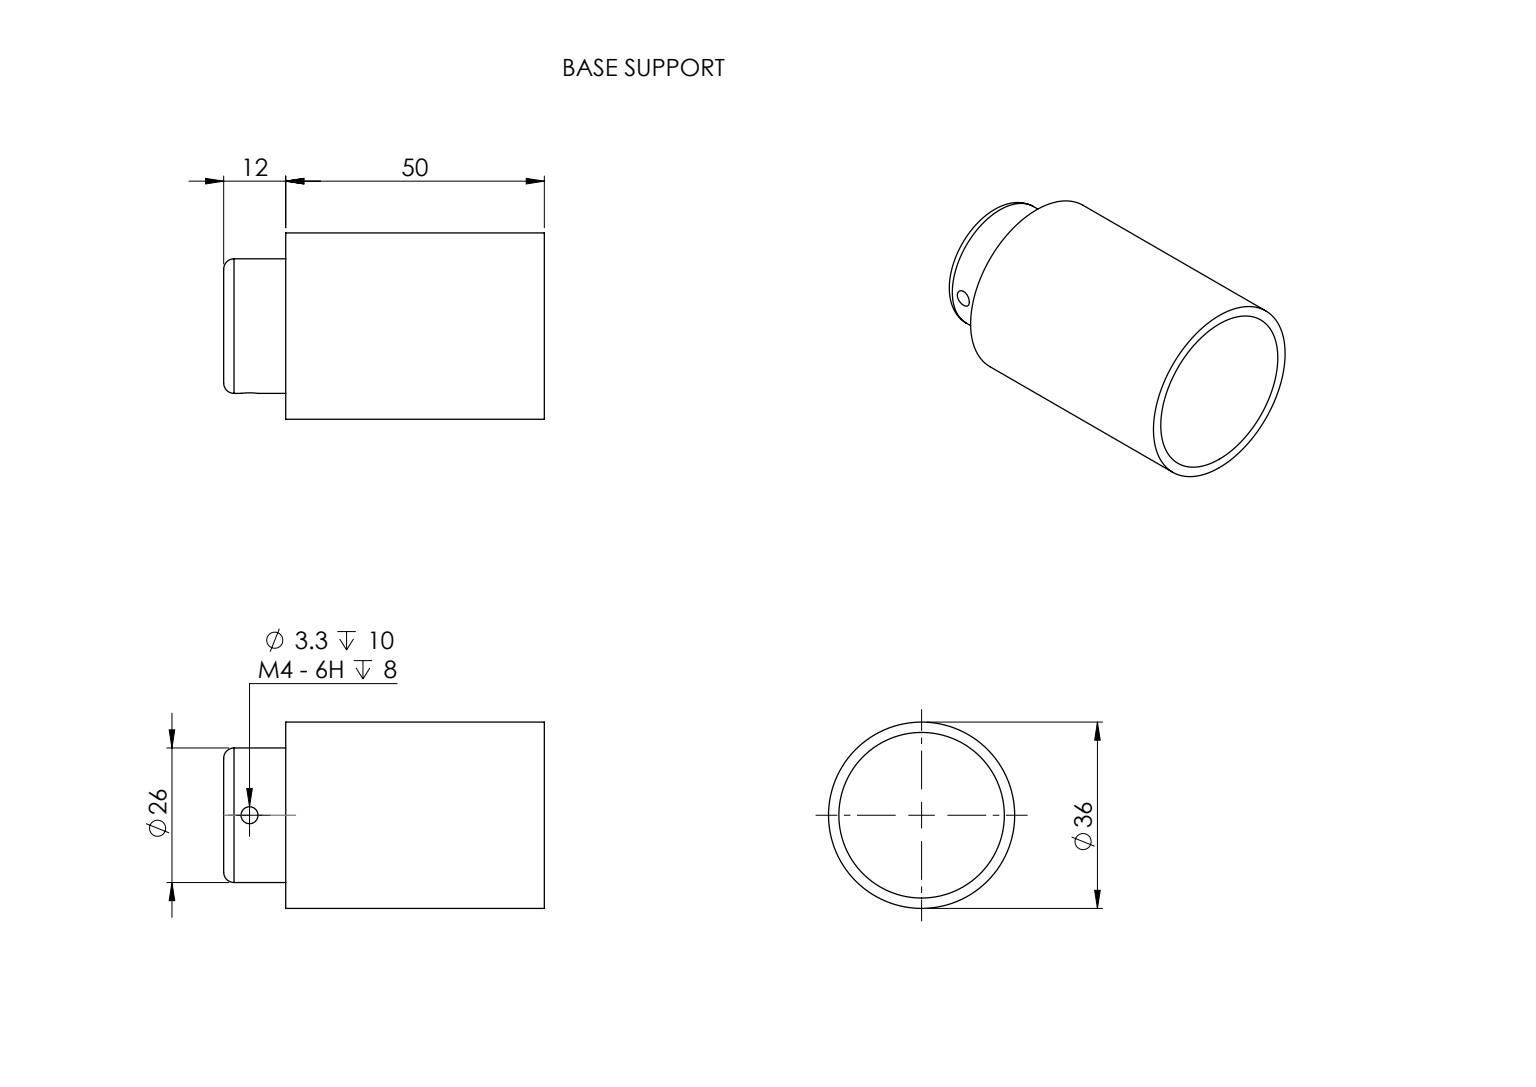
ISO-10303-21;
HEADER;
FILE_DESCRIPTION (('STEP AP214'),
    '1' );
FILE_NAME ('base support.step',
    '2026-10-08T13:22:57',
    ( '' ),
    ( '' ),
    'SwSTEP 2.0',
    'SolidWorks 2026',
    '' );
FILE_SCHEMA (( 'AUTOMOTIVE_DESIGN' ));
ENDSEC;

DATA;
#9=AXIS2_PLACEMENT_3D ( 'NONE', #1726, #4047, #111 ) ;
#21=CARTESIAN_POINT ( 'NONE',  ( -170.0000000000000284, -1.448262861947153525E-15, 0.000000000000000000 ) ) ;
#44=ORIENTED_EDGE ( 'NONE', *, *, #5565, .F. ) ;
#74=EDGE_CURVE ( 'NONE', #951, #9116, #2667, .T. ) ;
#106=CARTESIAN_POINT ( 'NONE',  ( -163.3500000000000796, 0.1091377801384209867, 13.00000000000000178 ) ) ;
#111=DIRECTION ( 'NONE',  ( 1.000000000000000000, 0.000000000000000000, 0.000000000000000000 ) ) ;
#152=FACE_BOUND ( 'NONE', #612, .T. ) ;
#164=AXIS2_PLACEMENT_3D ( 'NONE', #7046, #7979, #7201 ) ;
#171=CIRCLE ( 'NONE', #2486, 11.00000000000000355 ) ;
#181=CIRCLE ( 'NONE', #5941, 18.00000000000000355 ) ;
#189=AXIS2_PLACEMENT_3D ( 'NONE', #6209, #7825, #5544 ) ;
#214=CARTESIAN_POINT ( 'NONE',  ( -163.5173699842553390, 0.7321227054117522837, 12.97975339917165805 ) ) ;
#245=CARTESIAN_POINT ( 'NONE',  ( 0.000000000000000000, 0.000000000000000000, 0.000000000000000000 ) ) ;
#310=EDGE_CURVE ( 'NONE', #9116, #951, #8435, .T. ) ;
#313=EDGE_LOOP ( 'NONE', ( #4589, #4798, #9873, #8476 ) ) ;
#325=CARTESIAN_POINT ( 'NONE',  ( -165.4284909017565326, -1.597016366731424553, 12.90154986763612577 ) ) ;
#348=VECTOR ( 'NONE', #8424, 1000.000000000000000 ) ;
#354=ORIENTED_EDGE ( 'NONE', *, *, #6522, .T. ) ;
#366=LINE ( 'NONE', #6691, #7331 ) ;
#380=DIRECTION ( 'NONE',  ( 0.000000000000000000, 1.000000000000000000, 0.000000000000000000 ) ) ;
#388=ORIENTED_EDGE ( 'NONE', *, *, #1909, .T. ) ;
#394=ADVANCED_FACE ( 'NONE', ( #8448 ), #10092, .T. ) ;
#413=EDGE_LOOP ( 'NONE', ( #2584, #9697, #9041, #6358 ) ) ;
#416=CARTESIAN_POINT ( 'NONE',  ( -166.6500000000000341, -1.532656777835077474E-15, 13.00000000000000355 ) ) ;
#449=AXIS2_PLACEMENT_3D ( 'NONE', #4004, #8752, #7976 ) ;
#451=APPLICATION_CONTEXT ( 'automotive_design' ) ;
#472=DIRECTION ( 'NONE',  ( -1.000000000000000000, -1.387778780781445676E-16, -0.000000000000000000 ) ) ;
#503=VERTEX_POINT ( 'NONE', #9443 ) ;
#520=CARTESIAN_POINT ( 'NONE',  ( -108.0000000000000426, 18.00000000000000355, 0.000000000000000000 ) ) ;
#545=CIRCLE ( 'NONE', #4999, 13.00000000000000533 ) ;
#590=DIRECTION ( 'NONE',  ( -0.000000000000000000, 0.000000000000000000, -1.000000000000000000 ) ) ;
#607=ORIENTED_EDGE ( 'NONE', *, *, #8566, .T. ) ;
#609=ADVANCED_FACE ( 'NONE', ( #8706 ), #801, .F. ) ;
#612=EDGE_LOOP ( 'NONE', ( #1014, #1623 ) ) ;
#656=CARTESIAN_POINT ( 'NONE',  ( -158.0000000000000284, -16.00000000000000355, 0.000000000000000000 ) ) ;
#662=EDGE_LOOP ( 'NONE', ( #7898, #847, #3202, #5619 ) ) ;
#685=LINE ( 'NONE', #2124, #348 ) ;
#726=ORIENTED_EDGE ( 'NONE', *, *, #882, .T. ) ;
#781=FACE_OUTER_BOUND ( 'NONE', #3740, .T. ) ;
#801=CYLINDRICAL_SURFACE ( 'NONE', #164, 15.99999999999999645 ) ;
#830=CARTESIAN_POINT ( 'NONE',  ( -158.0000000000000284, -6.938893903907228378E-15, 0.000000000000000000 ) ) ;
#833=CIRCLE ( 'NONE', #9, 1.649999999999984812 ) ;
#838=CARTESIAN_POINT ( 'NONE',  ( -165.2165827598522867, 1.639280964940008856, 12.89624789671500515 ) ) ;
#847=ORIENTED_EDGE ( 'NONE', *, *, #5286, .T. ) ;
#860=COLOUR_RGB ( '', 0.31764706, 0.68627451, 0.89019608) ;
#882=EDGE_CURVE ( 'NONE', #6987, #9116, #2598, .T. ) ;
#906=CARTESIAN_POINT ( 'NONE',  ( -164.5737606474697543, -1.597621038677511818, 12.90147476577599406 ) ) ;
#943=CARTESIAN_POINT ( 'NONE',  ( -165.4282927514613277, 1.597095956079517709, 12.90154007871212194 ) ) ;
#951=VERTEX_POINT ( 'NONE', #6970 ) ;
#978=ORIENTED_EDGE ( 'NONE', *, *, #8970, .F. ) ;
#992=ADVANCED_FACE ( 'NONE', ( #4599 ), #10132, .F. ) ;
#1004=CIRCLE ( 'NONE', #6592, 11.00000000000000355 ) ;
#1006=CIRCLE ( 'NONE', #2647, 2.000000000000001776 ) ;
#1014=ORIENTED_EDGE ( 'NONE', *, *, #5317, .T. ) ;
#1057=DIRECTION ( 'NONE',  ( -0.000000000000000000, -0.000000000000000000, 1.000000000000000000 ) ) ;
#1095=DIRECTION ( 'NONE',  ( -0.8571673007021101132, 1.049727191138615984E-16, 0.5150380749100580413 ) ) ;
#1118=CARTESIAN_POINT ( 'NONE',  ( -165.0000000000000284, -1.734723475976807094E-15, 3.000000000000002665 ) ) ;
#1188=CARTESIAN_POINT ( 'NONE',  ( -166.6500000000000341, 0.1077421301470921078, 13.00000000000000711 ) ) ;
#1205=CIRCLE ( 'NONE', #4016, 13.00000000000000533 ) ;
#1223=SURFACE_STYLE_FILL_AREA ( #2208 ) ;
#1248=CARTESIAN_POINT ( 'NONE',  ( -168.0000000000000284, -2.363368035607157783E-15, 0.000000000000000000 ) ) ;
#1261=B_SPLINE_CURVE_WITH_KNOTS ( 'NONE', 3,
 ( #8909, #4251, #3421, #4979, #3329, #8862, #1682, #6465, #3471, #2447, #325, #1775, #9539, #5592, #4825, #906, #4928, #4053, #7200, #8075, #6814, #5273, #2846, #2741, #3570, #4300 ),
 .UNSPECIFIED., .F., .F.,
 ( 4, 2, 2, 2, 2, 2, 2, 2, 2, 2, 2, 2, 4 ),
 ( 0.005163858345264566406, 0.005809185821787722637, 0.006454513298310878000, 0.006777177036572426191, 0.007099840774833974383, 0.007422504513095522574, 0.007745168251357070766, 0.008067831989618618957, 0.008390495727880167148, 0.008713159466141713605, 0.009035823204403263531, 0.009681150680926300933, 0.01032647815744933834 ),
 .UNSPECIFIED. ) ;
#1268=( LENGTH_UNIT ( ) NAMED_UNIT ( * ) SI_UNIT ( .MILLI., .METRE. ) );
#1288=CARTESIAN_POINT ( 'NONE',  ( -166.2435802567831331, 1.089887640161022464, 12.95446314200367155 ) ) ;
#1302=CARTESIAN_POINT ( 'NONE',  ( -158.0000000000000284, -6.938893903907228378E-15, 0.000000000000000000 ) ) ;
#1352=( GEOMETRIC_REPRESENTATION_CONTEXT ( 3 ) GLOBAL_UNCERTAINTY_ASSIGNED_CONTEXT ( ( #4119 ) ) GLOBAL_UNIT_ASSIGNED_CONTEXT ( ( #8397, #9910, #4533 ) ) REPRESENTATION_CONTEXT ( 'NONE', 'WORKASPACE' ) );
#1420=DIRECTION ( 'NONE',  ( 0.000000000000000000, -1.000000000000000000, 0.000000000000000000 ) ) ;
#1438=EDGE_LOOP ( 'NONE', ( #8309, #6120, #4912 ) ) ;
#1508=EDGE_CURVE ( 'NONE', #3127, #9396, #1750, .T. ) ;
#1510=ADVANCED_FACE ( 'NONE', ( #9562 ), #7923, .T. ) ;
#1563=AXIS2_PLACEMENT_3D ( 'NONE', #520, #6802, #6597 ) ;
#1613=VERTEX_POINT ( 'NONE', #2001 ) ;
#1616=CARTESIAN_POINT ( 'NONE',  ( -168.0000000000000284, -2.363368035607157783E-15, 0.000000000000000000 ) ) ;
#1623=ORIENTED_EDGE ( 'NONE', *, *, #5748, .T. ) ;
#1637=CARTESIAN_POINT ( 'NONE',  ( -170.0000000000000284, -1.448262861947153525E-15, 0.000000000000000000 ) ) ;
#1666=FACE_OUTER_BOUND ( 'NONE', #313, .T. ) ;
#1676=AXIS2_PLACEMENT_3D ( 'NONE', #7871, #8656, #7781 ) ;
#1682=CARTESIAN_POINT ( 'NONE',  ( -166.0067307485407184, -1.311714535335565923, 12.93379411699749681 ) ) ;
#1720=CARTESIAN_POINT ( 'NONE',  ( -163.4027093359710534, 0.4274795813385452448, 12.99339846045314850 ) ) ;
#1726=CARTESIAN_POINT ( 'NONE',  ( -165.0000000000000284, -1.734723475976807094E-15, 3.000000000000002665 ) ) ;
#1750=LINE ( 'NONE', #5814, #7591 ) ;
#1763=LINE ( 'NONE', #9577, #3701 ) ;
#1775=CARTESIAN_POINT ( 'NONE',  ( -165.2175649311437837, -1.639125141419205622, 12.89626763964974465 ) ) ;
#1783=EDGE_CURVE ( 'NONE', #503, #6536, #171, .T. ) ;
#1826=AXIS2_PLACEMENT_3D ( 'NONE', #4668, #5385, #3735 ) ;
#1863=ORIENTED_EDGE ( 'NONE', *, *, #1508, .T. ) ;
#1866=CARTESIAN_POINT ( 'NONE',  ( -164.7839123519666487, 1.649920478573665195, 12.89487349378784664 ) ) ;
#1870=EDGE_CURVE ( 'NONE', #5718, #951, #10115, .T. ) ;
#1871=DIRECTION ( 'NONE',  ( 0.000000000000000000, -1.000000000000000000, 0.000000000000000000 ) ) ;
#1881=DIRECTION ( 'NONE',  ( -5.603403109029596495E-32, -1.224646799147353207E-16, 1.000000000000000000 ) ) ;
#1905=ORIENTED_EDGE ( 'NONE', *, *, #6467, .T. ) ;
#1909=EDGE_CURVE ( 'NONE', #6987, #5718, #9429, .T. ) ;
#1982=ORIENTED_EDGE ( 'NONE', *, *, #310, .T. ) ;
#1988=DIRECTION ( 'NONE',  ( -4.575525868300071581E-16, -1.000000000000000000, 0.000000000000000000 ) ) ;
#1995=VECTOR ( 'NONE', #4731, 1000.000000000000000 ) ;
#2001=CARTESIAN_POINT ( 'NONE',  ( -158.0000000000000284, -13.00000000000001066, 1.592040838891559884E-15 ) ) ;
#2014=CARTESIAN_POINT ( 'NONE',  ( -166.5969417738770346, 0.4288646725500943613, 12.99335536005336955 ) ) ;
#2060=EDGE_CURVE ( 'NONE', #6536, #503, #1004, .T. ) ;
#2065=CARTESIAN_POINT ( 'NONE',  ( -170.0000000000000284, 11.00000000000000178, 1.469576158976824539E-15 ) ) ;
#2097=( NAMED_UNIT ( * ) SI_UNIT ( $, .STERADIAN. ) SOLID_ANGLE_UNIT ( ) );
#2118=LINE ( 'NONE', #9875, #8996 ) ;
#2124=CARTESIAN_POINT ( 'NONE',  ( -158.0000000000000284, -13.00000000000001066, 1.592040838891559490E-15 ) ) ;
#2144=CARTESIAN_POINT ( 'NONE',  ( -158.0000000000000284, -6.938893903907228378E-15, 0.000000000000000000 ) ) ;
#2145=FACE_OUTER_BOUND ( 'NONE', #4650, .T. ) ;
#2151=SURFACE_STYLE_USAGE ( .BOTH. , #8508 ) ;
#2185=DIRECTION ( 'NONE',  ( -0.000000000000000000, -0.000000000000000000, 1.000000000000000000 ) ) ;
#2202=DIRECTION ( 'NONE',  ( 0.000000000000000000, -1.000000000000000000, 0.000000000000000000 ) ) ;
#2208=FILL_AREA_STYLE ('',( #6781 ) ) ;
#2239=FACE_OUTER_BOUND ( 'NONE', #413, .T. ) ;
#2264=ADVANCED_FACE ( 'NONE', ( #8085 ), #5129, .F. ) ;
#2310=DIRECTION ( 'NONE',  ( 0.000000000000000000, -1.000000000000000000, 0.000000000000000000 ) ) ;
#2359=CIRCLE ( 'NONE', #2542, 13.00000000000000355 ) ;
#2364=SHAPE_DEFINITION_REPRESENTATION ( #5902, #5586 ) ;
#2435=CARTESIAN_POINT ( 'NONE',  ( -165.8275777035124747, 1.431488817417934101, 12.92108529057806798 ) ) ;
#2447=CARTESIAN_POINT ( 'NONE',  ( -165.5332536431789094, -1.565195349311612416, 12.90549919778201904 ) ) ;
#2477=VECTOR ( 'NONE', #8016, 1000.000000000000000 ) ;
#2482=CARTESIAN_POINT ( 'NONE',  ( -163.5680690899785930, 0.8268589710946947502, 12.97398861359800115 ) ) ;
#2486=AXIS2_PLACEMENT_3D ( 'NONE', #1637, #10163, #4736 ) ;
#2498=CARTESIAN_POINT ( 'NONE',  ( -158.0000000000000284, -6.938893903907228378E-15, 0.000000000000000000 ) ) ;
#2524=VERTEX_POINT ( 'NONE', #9898 ) ;
#2542=AXIS2_PLACEMENT_3D ( 'NONE', #1616, #4613, #6093 ) ;
#2584=ORIENTED_EDGE ( 'NONE', *, *, #9584, .F. ) ;
#2595=FACE_BOUND ( 'NONE', #7310, .T. ) ;
#2598=LINE ( 'NONE', #3472, #5924 ) ;
#2630=FACE_OUTER_BOUND ( 'NONE', #9178, .T. ) ;
#2643=DIRECTION ( 'NONE',  ( 1.000000000000000000, -4.575525868300071581E-16, -0.000000000000000000 ) ) ;
#2647=AXIS2_PLACEMENT_3D ( 'NONE', #3893, #590, #4517 ) ;
#2667=CIRCLE ( 'NONE', #8620, 18.00000000000000355 ) ;
#2681=CYLINDRICAL_SURFACE ( 'NONE', #7208, 18.00000000000000355 ) ;
#2695=CARTESIAN_POINT ( 'NONE',  ( -168.0000000000000284, 13.00000000000000178, 0.000000000000000000 ) ) ;
#2705=ORIENTED_EDGE ( 'NONE', *, *, #2060, .F. ) ;
#2734=FACE_OUTER_BOUND ( 'NONE', #1438, .T. ) ;
#2741=CARTESIAN_POINT ( 'NONE',  ( -163.3939431418218646, -0.4350255360096275670, 12.99423751676100558 ) ) ;
#2781=EDGE_CURVE ( 'NONE', #9967, #8413, #8938, .T. ) ;
#2846=CARTESIAN_POINT ( 'NONE',  ( -163.5589117782047595, -0.8318236505920658663, 12.97488054948080993 ) ) ;
#2886=FACE_OUTER_BOUND ( 'NONE', #8049, .T. ) ;
#2903=EDGE_CURVE ( 'NONE', #10190, #9396, #6449, .T. ) ;
#2943=DIRECTION ( 'NONE',  ( 1.000000000000000000, 0.000000000000000000, 0.000000000000000000 ) ) ;
#2949=CARTESIAN_POINT ( 'NONE',  ( -166.6500000000000341, -1.532656777835077474E-15, 13.00000000000000355 ) ) ;
#2953=CARTESIAN_POINT ( 'NONE',  ( -108.0000000000000426, 15.99999999999999289, 1.959434878635764737E-15 ) ) ;
#3094=CYLINDRICAL_SURFACE ( 'NONE', #3255, 1.649999999999984812 ) ;
#3122=CARTESIAN_POINT ( 'NONE',  ( -168.0000000000000284, -13.00000000000000533, 1.592040838891559490E-15 ) ) ;
#3127=VERTEX_POINT ( 'NONE', #6508 ) ;
#3143=ADVANCED_FACE ( 'NONE', ( #2595, #5791 ), #3419, .T. ) ;
#3152=STYLED_ITEM ( 'NONE', ( #9506 ), #7057 ) ;
#3153=AXIS2_PLACEMENT_3D ( 'NONE', #5901, #9077, #1988 ) ;
#3161=( GEOMETRIC_REPRESENTATION_CONTEXT ( 3 ) GLOBAL_UNCERTAINTY_ASSIGNED_CONTEXT ( ( #8141 ) ) GLOBAL_UNIT_ASSIGNED_CONTEXT ( ( #1268, #9235, #2097 ) ) REPRESENTATION_CONTEXT ( 'NONE', 'WORKASPACE' ) );
#3190=AXIS2_PLACEMENT_3D ( 'NONE', #5290, #5144, #8391 ) ;
#3202=ORIENTED_EDGE ( 'NONE', *, *, #1783, .F. ) ;
#3204=EDGE_CURVE ( 'NONE', #9396, #6730, #9685, .T. ) ;
#3218=LINE ( 'NONE', #4096, #2477 ) ;
#3255=AXIS2_PLACEMENT_3D ( 'NONE', #8526, #3774, #6906 ) ;
#3272=DIRECTION ( 'NONE',  ( -1.000000000000000000, -1.387778780781445676E-16, -0.000000000000000000 ) ) ;
#3310=AXIS2_PLACEMENT_3D ( 'NONE', #10146, #8494, #1420 ) ;
#3329=CARTESIAN_POINT ( 'NONE',  ( -166.3194911921033849, -1.013757292147143385, 12.96131341066429954 ) ) ;
#3342=FILL_AREA_STYLE_COLOUR ( '', #7114 ) ;
#3394=CARTESIAN_POINT ( 'NONE',  ( -166.6500000000000341, -1.532656754117495520E-15, 3.000000000000002665 ) ) ;
#3397=CARTESIAN_POINT ( 'NONE',  ( -168.0000000000000284, -2.363368035607170010E-15, 0.000000000000000000 ) ) ;
#3411=CARTESIAN_POINT ( 'NONE',  ( -164.1695521934695989, 1.441888585351695395, 12.92005519273647707 ) ) ;
#3419=CYLINDRICAL_SURFACE ( 'NONE', #449, 13.00000000000000355 ) ;
#3421=CARTESIAN_POINT ( 'NONE',  ( -166.6066941517921123, -0.4327006227615173839, 12.99431788236279139 ) ) ;
#3445=EDGE_LOOP ( 'NONE', ( #8575, #3826, #7606, #9478 ) ) ;
#3451=ORIENTED_EDGE ( 'NONE', *, *, #5975, .F. ) ;
#3468=VERTEX_POINT ( 'NONE', #2695 ) ;
#3471=CARTESIAN_POINT ( 'NONE',  ( -165.7329923747223859, -1.482200427765804296, 12.91529434110542240 ) ) ;
#3472=CARTESIAN_POINT ( 'NONE',  ( -158.0000000000000284, -18.00000000000001066, 0.000000000000000000 ) ) ;
#3565=CARTESIAN_POINT ( 'NONE',  ( -108.0000000000000426, 0.000000000000000000, 0.000000000000000000 ) ) ;
#3570=CARTESIAN_POINT ( 'NONE',  ( -163.3500000000000796, -0.2182232076591351377, 13.00000000000000533 ) ) ;
#3598=ORIENTED_EDGE ( 'NONE', *, *, #1870, .F. ) ;
#3646=ADVANCED_FACE ( 'NONE', ( #2630 ), #2681, .T. ) ;
#3689=ORIENTED_EDGE ( 'NONE', *, *, #3204, .F. ) ;
#3701=VECTOR ( 'NONE', #4141, 1000.000000000000000 ) ;
#3709=CARTESIAN_POINT ( 'NONE',  ( -108.0000000000000426, -18.00000000000000355, 0.000000000000000000 ) ) ;
#3735=DIRECTION ( 'NONE',  ( 0.000000000000000000, -1.000000000000000000, 0.000000000000000000 ) ) ;
#3740=EDGE_LOOP ( 'NONE', ( #1982, #8387 ) ) ;
#3774=DIRECTION ( 'NONE',  ( -0.000000000000000000, -0.000000000000000000, 1.000000000000000000 ) ) ;
#3826=ORIENTED_EDGE ( 'NONE', *, *, #9652, .T. ) ;
#3836=ADVANCED_FACE ( 'NONE', ( #5258 ), #3094, .F. ) ;
#3842=CARTESIAN_POINT ( 'NONE',  ( -156.0000000000000284, -16.00000000000000711, 0.000000000000000000 ) ) ;
#3893=CARTESIAN_POINT ( 'NONE',  ( -168.0000000000000284, -11.00000000000000533, 0.000000000000000000 ) ) ;
#3977=AXIS2_PLACEMENT_3D ( 'NONE', #1118, #5704, #7363 ) ;
#3986=PLANE ( 'NONE',  #7782 ) ;
#3988=AXIS2_PLACEMENT_3D ( 'NONE', #5116, #2185, #2943 ) ;
#3995=AXIS2_PLACEMENT_3D ( 'NONE', #245, #8930, #7419 ) ;
#4004=CARTESIAN_POINT ( 'NONE',  ( -158.0000000000000284, -6.938893903907228378E-15, 0.000000000000000000 ) ) ;
#4016=AXIS2_PLACEMENT_3D ( 'NONE', #1302, #9216, #380 ) ;
#4044=CARTESIAN_POINT ( 'NONE',  ( -158.0000000000000284, -6.938893903907228378E-15, 0.000000000000000000 ) ) ;
#4047=DIRECTION ( 'NONE',  ( -0.000000000000000000, -0.000000000000000000, 1.000000000000000000 ) ) ;
#4053=CARTESIAN_POINT ( 'NONE',  ( -164.2691053559693728, -1.483232571104735609, 12.91517534017533109 ) ) ;
#4089=CARTESIAN_POINT ( 'NONE',  ( -165.5312037683856943, 1.565894570282060583, 12.90541399993123228 ) ) ;
#4096=CARTESIAN_POINT ( 'NONE',  ( -158.0000000000000284, 15.99999999999998934, 1.959434878635764737E-15 ) ) ;
#4119=UNCERTAINTY_MEASURE_WITH_UNIT (LENGTH_MEASURE( 1.000000000000000082E-05 ), #8397, 'distance_accuracy_value', 'NONE');
#4141=DIRECTION ( 'NONE',  ( -0.000000000000000000, -0.000000000000000000, 1.000000000000000000 ) ) ;
#4144=AXIS2_PLACEMENT_3D ( 'NONE', #5292, #8449, #2202 ) ;
#4153=DIRECTION ( 'NONE',  ( 0.000000000000000000, -1.000000000000000000, -1.224646799147353454E-16 ) ) ;
#4192=DIRECTION ( 'NONE',  ( 1.000000000000000000, -4.575525868300071581E-16, -0.000000000000000000 ) ) ;
#4235=DIRECTION ( 'NONE',  ( 1.000000000000000000, -4.575525868300071581E-16, -0.000000000000000000 ) ) ;
#4251=CARTESIAN_POINT ( 'NONE',  ( -166.6500000000000057, -0.2154325771598549211, 13.00000000000000533 ) ) ;
#4275=EDGE_LOOP ( 'NONE', ( #5969, #1863, #9950 ) ) ;
#4300=CARTESIAN_POINT ( 'NONE',  ( -163.3500000000000512, -1.154202410357457390E-14, 13.00000000000000355 ) ) ;
#4301=VECTOR ( 'NONE', #6221, 1000.000000000000000 ) ;
#4312=ORIENTED_EDGE ( 'NONE', *, *, #74, .F. ) ;
#4337=CARTESIAN_POINT ( 'NONE',  ( -166.4312272284851986, 0.8280293812990602298, 12.97391163473193387 ) ) ;
#4379=ORIENTED_EDGE ( 'NONE', *, *, #1870, .T. ) ;
#4454=DIRECTION ( 'NONE',  ( 1.000000000000000000, -4.575525868300071581E-16, -0.000000000000000000 ) ) ;
#4486=STYLED_ITEM ( 'NONE', ( #5201 ), #8958 ) ;
#4517=DIRECTION ( 'NONE',  ( -1.000000000000000000, 0.000000000000000000, 0.000000000000000000 ) ) ;
#4533=( NAMED_UNIT ( * ) SI_UNIT ( $, .STERADIAN. ) SOLID_ANGLE_UNIT ( ) );
#4539=ORIENTED_EDGE ( 'NONE', *, *, #9349, .F. ) ;
#4541=DIRECTION ( 'NONE',  ( 0.000000000000000000, -1.000000000000000000, 0.000000000000000000 ) ) ;
#4573=EDGE_LOOP ( 'NONE', ( #7823, #3451, #5167, #2705 ) ) ;
#4585=SHAPE_REPRESENTATION_RELATIONSHIP ( 'NONE' , 'NONE' ,  #5586, #8958 ) ;
#4589=ORIENTED_EDGE ( 'NONE', *, *, #9652, .F. ) ;
#4599=FACE_OUTER_BOUND ( 'NONE', #9240, .T. ) ;
#4607=CARTESIAN_POINT ( 'NONE',  ( -156.0000000000000284, -6.938893903907228378E-15, 0.000000000000000000 ) ) ;
#4613=DIRECTION ( 'NONE',  ( 1.000000000000000000, -4.575525868300071581E-16, -0.000000000000000000 ) ) ;
#4650=EDGE_LOOP ( 'NONE', ( #388, #4379, #5159, #4762 ) ) ;
#4661=ORIENTED_EDGE ( 'NONE', *, *, #1909, .F. ) ;
#4668=CARTESIAN_POINT ( 'NONE',  ( -158.0000000000000284, -6.938893903907228378E-15, 0.000000000000000000 ) ) ;
#4731=DIRECTION ( 'NONE',  ( -1.000000000000000000, -1.387778780781445676E-16, -0.000000000000000000 ) ) ;
#4736=DIRECTION ( 'NONE',  ( 0.000000000000000000, -1.000000000000000000, 0.000000000000000000 ) ) ;
#4739=SURFACE_SIDE_STYLE ('',( #4940 ) ) ;
#4762=ORIENTED_EDGE ( 'NONE', *, *, #882, .F. ) ;
#4782=AXIS2_PLACEMENT_3D ( 'NONE', #2144, #5349, #5291 ) ;
#4789=AXIS2_PLACEMENT_3D ( 'NONE', #3397, #5617, #8837 ) ;
#4798=ORIENTED_EDGE ( 'NONE', *, *, #5975, .T. ) ;
#4814=ADVANCED_FACE ( 'NONE', ( #9900 ), #10001, .F. ) ;
#4815=CARTESIAN_POINT ( 'NONE',  ( -163.9856078553142709, 1.318997900831586856, 12.93381406529030642 ) ) ;
#4825=CARTESIAN_POINT ( 'NONE',  ( -164.7848126586117985, -1.639441178260655052, 12.89622722885275152 ) ) ;
#4842=AXIS2_PLACEMENT_3D ( 'NONE', #21, #6993, #8501 ) ;
#4866=CARTESIAN_POINT ( 'NONE',  ( -163.7574652328086131, 1.090948703523729746, 12.95436823472124566 ) ) ;
#4912=ORIENTED_EDGE ( 'NONE', *, *, #2903, .T. ) ;
#4928=CARTESIAN_POINT ( 'NONE',  ( -164.4688726891355088, -1.565914946704515254, 12.90541139627661593 ) ) ;
#4940=SURFACE_STYLE_FILL_AREA ( #9657 ) ;
#4964=CIRCLE ( 'NONE', #3310, 16.00000000000000000 ) ;
#4979=CARTESIAN_POINT ( 'NONE',  ( -166.4422304502845407, -0.8298597800914565559, 12.97500904825187540 ) ) ;
#4981=ADVANCED_FACE ( 'NONE', ( #5348 ), #5499, .T. ) ;
#4986=CLOSED_SHELL ( 'NONE', ( #3836, #9463, #394, #3143, #7435, #8404, #992, #609, #6555, #3646, #9871, #6343, #4981, #1510, #2264, #4814 ) ) ;
#4999=AXIS2_PLACEMENT_3D ( 'NONE', #2498, #2643, #8126 ) ;
#5014=CARTESIAN_POINT ( 'NONE',  ( -165.1071317273496959, 1.650039592648423259, 12.89485825219862569 ) ) ;
#5066=CARTESIAN_POINT ( 'NONE',  ( -163.3500000000000512, -1.734723475976807094E-15, 3.000000000000002665 ) ) ;
#5087=PRODUCT ( 'base support', 'base support', '', ( #10170 ) ) ;
#5088=B_SPLINE_CURVE_WITH_KNOTS ( 'NONE', 3,
 ( #7291, #106, #8802, #1720, #6351, #214, #2482, #5636, #4866, #4815, #3411, #6547, #1866, #5014, #838, #943, #4089, #9529, #2435, #5581, #7965, #1288, #7387, #4337, #7440, #9104, #2014, #8265, #1188, #416 ),
 .UNSPECIFIED., .F., .F.,
 ( 4, 2, 2, 2, 2, 2, 2, 2, 2, 2, 2, 2, 2, 2, 4 ),
 ( 6.815973429434667561E-18, 0.0003227411465790211431, 0.0006454822931580354558, 0.0009682234397370497684, 0.001290964586316063973, 0.001936446879474092598, 0.002581929172632121440, 0.002904670319211177278, 0.003227411465790232682, 0.003550152612369288519, 0.003872893758948343923, 0.004195634905527399761, 0.004518376052106455598, 0.004841117198685510568, 0.005163858345264566406 ),
 .UNSPECIFIED. ) ;
#5116=CARTESIAN_POINT ( 'NONE',  ( -165.0000000000000284, -1.734723475976807094E-15, 3.000000000000002665 ) ) ;
#5129=CONICAL_SURFACE ( 'NONE', #3977, 1.649999999999984812, 1.029744258676650093 ) ;
#5144=DIRECTION ( 'NONE',  ( -0.000000000000000000, -0.000000000000000000, 1.000000000000000000 ) ) ;
#5159=ORIENTED_EDGE ( 'NONE', *, *, #310, .F. ) ;
#5167=ORIENTED_EDGE ( 'NONE', *, *, #8383, .T. ) ;
#5201=PRESENTATION_STYLE_ASSIGNMENT (( #2151 ) ) ;
#5216=PLANE ( 'NONE',  #1563 ) ;
#5249=CARTESIAN_POINT ( 'NONE',  ( -158.0000000000000284, -6.938893903907228378E-15, 0.000000000000000000 ) ) ;
#5258=FACE_OUTER_BOUND ( 'NONE', #9916, .T. ) ;
#5273=CARTESIAN_POINT ( 'NONE',  ( -163.6819620139764595, -1.015622990690433936, 12.96116402481652408 ) ) ;
#5286=EDGE_CURVE ( 'NONE', #3468, #6536, #5331, .T. ) ;
#5288=CIRCLE ( 'NONE', #9770, 16.00000000000000000 ) ;
#5290=CARTESIAN_POINT ( 'NONE',  ( -165.0000000000000284, -1.734723475976807094E-15, 13.00000000000000355 ) ) ;
#5291=DIRECTION ( 'NONE',  ( 0.000000000000000000, -1.000000000000000000, 0.000000000000000000 ) ) ;
#5292=CARTESIAN_POINT ( 'NONE',  ( -158.0000000000000284, -6.938893903907228378E-15, 0.000000000000000000 ) ) ;
#5317=EDGE_CURVE ( 'NONE', #2524, #1613, #545, .T. ) ;
#5331=CIRCLE ( 'NONE', #6974, 2.000000000000000000 ) ;
#5348=FACE_OUTER_BOUND ( 'NONE', #8939, .T. ) ;
#5349=DIRECTION ( 'NONE',  ( -1.000000000000000000, -1.387778780781445676E-16, -0.000000000000000000 ) ) ;
#5385=DIRECTION ( 'NONE',  ( -1.000000000000000000, -1.387778780781445676E-16, -0.000000000000000000 ) ) ;
#5418=ORIENTED_EDGE ( 'NONE', *, *, #2060, .T. ) ;
#5499=PLANE ( 'NONE',  #4842 ) ;
#5509=DIRECTION ( 'NONE',  ( -1.000000000000000000, 4.575525868300071581E-16, 0.000000000000000000 ) ) ;
#5531=EDGE_LOOP ( 'NONE', ( #8199, #8633 ) ) ;
#5544=DIRECTION ( 'NONE',  ( 1.000000000000000000, 0.000000000000000000, 0.000000000000000000 ) ) ;
#5556=CARTESIAN_POINT ( 'NONE',  ( -158.0000000000000284, 17.99999999999999645, 2.204364238465235822E-15 ) ) ;
#5565=EDGE_CURVE ( 'NONE', #5950, #6730, #1261, .T. ) ;
#5581=CARTESIAN_POINT ( 'NONE',  ( -166.0062384261120769, 1.312070622931204689, 12.93375722677777340 ) ) ;
#5586=SHAPE_REPRESENTATION ( 'base support', ( #3995 ), #3161 ) ;
#5592=CARTESIAN_POINT ( 'NONE',  ( -164.8920828308066859, -1.650077165904365373, 12.89485344440482173 ) ) ;
#5604=PRODUCT_DEFINITION ( 'UNKNOWN', '', #7888, #7116 ) ;
#5617=DIRECTION ( 'NONE',  ( -1.000000000000000000, 4.575525868300071581E-16, 0.000000000000000000 ) ) ;
#5619=ORIENTED_EDGE ( 'NONE', *, *, #8383, .F. ) ;
#5629=DIRECTION ( 'NONE',  ( 1.000000000000000000, 1.387778780781445676E-16, 0.000000000000000000 ) ) ;
#5636=CARTESIAN_POINT ( 'NONE',  ( -163.6878309682295765, 1.006148260057784238, 12.96131713918894235 ) ) ;
#5704=DIRECTION ( 'NONE',  ( -0.000000000000000000, -0.000000000000000000, 1.000000000000000000 ) ) ;
#5714=DIRECTION ( 'NONE',  ( 0.8571673007021101132, 0.000000000000000000, 0.5150380749100580413 ) ) ;
#5718=VERTEX_POINT ( 'NONE', #7669 ) ;
#5748=EDGE_CURVE ( 'NONE', #1613, #2524, #1205, .T. ) ;
#5756=UNCERTAINTY_MEASURE_WITH_UNIT (LENGTH_MEASURE( 1.000000000000000082E-05 ), #7886, 'distance_accuracy_value', 'NONE');
#5778=DIRECTION ( 'NONE',  ( 0.000000000000000000, -1.000000000000000000, 0.000000000000000000 ) ) ;
#5791=FACE_OUTER_BOUND ( 'NONE', #3445, .T. ) ;
#5814=CARTESIAN_POINT ( 'NONE',  ( -163.3500000000000512, -1.734723475976807094E-15, 3.000000000000002665 ) ) ;
#5870=VECTOR ( 'NONE', #1057, 1000.000000000000000 ) ;
#5874=CARTESIAN_POINT ( 'NONE',  ( -158.0000000000000284, -6.938893903907228378E-15, 0.000000000000000000 ) ) ;
#5895=ORIENTED_EDGE ( 'NONE', *, *, #6467, .F. ) ;
#5901=CARTESIAN_POINT ( 'NONE',  ( -168.0000000000000284, -2.363368035607170010E-15, 0.000000000000000000 ) ) ;
#5902=PRODUCT_DEFINITION_SHAPE ( 'NONE', 'NONE',  #5604 ) ;
#5911=EDGE_CURVE ( 'NONE', #3468, #7869, #7670, .T. ) ;
#5924=VECTOR ( 'NONE', #3272, 1000.000000000000000 ) ;
#5941=AXIS2_PLACEMENT_3D ( 'NONE', #3565, #7496, #1871 ) ;
#5950=VERTEX_POINT ( 'NONE', #2949 ) ;
#5969=ORIENTED_EDGE ( 'NONE', *, *, #6565, .F. ) ;
#5975=EDGE_CURVE ( 'NONE', #7869, #3468, #2359, .T. ) ;
#5977=VERTEX_POINT ( 'NONE', #3842 ) ;
#5999=EDGE_LOOP ( 'NONE', ( #7068, #8364, #9837, #607 ) ) ;
#6032=CARTESIAN_POINT ( 'NONE',  ( -108.0000000000000426, 0.000000000000000000, 0.000000000000000000 ) ) ;
#6054=CYLINDRICAL_SURFACE ( 'NONE', #4144, 18.00000000000000355 ) ;
#6093=DIRECTION ( 'NONE',  ( 0.000000000000000000, -1.000000000000000000, 0.000000000000000000 ) ) ;
#6120=ORIENTED_EDGE ( 'NONE', *, *, #6565, .T. ) ;
#6209=CARTESIAN_POINT ( 'NONE',  ( -165.0000000000000284, -1.734723475976807094E-15, 3.000000000000002665 ) ) ;
#6221=DIRECTION ( 'NONE',  ( -1.000000000000000000, -1.387778780781445676E-16, -0.000000000000000000 ) ) ;
#6324=SURFACE_STYLE_USAGE ( .BOTH. , #4739 ) ;
#6335=ORIENTED_EDGE ( 'NONE', *, *, #5565, .T. ) ;
#6343=ADVANCED_FACE ( 'NONE', ( #1666 ), #7140, .T. ) ;
#6344=DIRECTION ( 'NONE',  ( -1.387778780781445676E-16, 1.000000000000000000, 0.000000000000000000 ) ) ;
#6351=CARTESIAN_POINT ( 'NONE',  ( -163.4344937688939865, 0.5323397972486557661, 12.98948098652724603 ) ) ;
#6358=ORIENTED_EDGE ( 'NONE', *, *, #7789, .F. ) ;
#6410=CARTESIAN_POINT ( 'NONE',  ( -163.3500000000000512, -1.734723475976807094E-15, 13.00000000000000355 ) ) ;
#6449=CIRCLE ( 'NONE', #189, 1.649999999999984812 ) ;
#6465=CARTESIAN_POINT ( 'NONE',  ( -165.8276565213533900, -1.431463064465520851, 12.92108891611541566 ) ) ;
#6467=EDGE_CURVE ( 'NONE', #10190, #5950, #1763, .T. ) ;
#6508=CARTESIAN_POINT ( 'NONE',  ( -165.0000000000000284, -1.734723475976807094E-15, 2.008579978604527305 ) ) ;
#6522=EDGE_CURVE ( 'NONE', #6730, #5950, #5088, .T. ) ;
#6536=VERTEX_POINT ( 'NONE', #2065 ) ;
#6547=CARTESIAN_POINT ( 'NONE',  ( -164.5666002992762458, 1.606502708168054738, 12.90062083485027777 ) ) ;
#6555=ADVANCED_FACE ( 'NONE', ( #2886, #8160 ), #5216, .F. ) ;
#6565=EDGE_CURVE ( 'NONE', #3127, #10190, #366, .T. ) ;
#6592=AXIS2_PLACEMENT_3D ( 'NONE', #8617, #5509, #7795 ) ;
#6597=DIRECTION ( 'NONE',  ( 1.387778780781445676E-16, -1.000000000000000000, 0.000000000000000000 ) ) ;
#6620=EDGE_CURVE ( 'NONE', #3468, #2524, #2118, .T. ) ;
#6633=ORIENTED_EDGE ( 'NONE', *, *, #9306, .F. ) ;
#6642=EDGE_LOOP ( 'NONE', ( #5895, #978, #9726, #354 ) ) ;
#6649=CARTESIAN_POINT ( 'NONE',  ( -156.0000000000000284, -6.661338147750945553E-15, 0.000000000000000000 ) ) ;
#6691=CARTESIAN_POINT ( 'NONE',  ( -166.6500000000000341, -1.532656754117495520E-15, 3.000000000000002665 ) ) ;
#6730=VERTEX_POINT ( 'NONE', #9158 ) ;
#6744=DIRECTION ( 'NONE',  ( 0.000000000000000000, -1.000000000000000000, 0.000000000000000000 ) ) ;
#6756=AXIS2_PLACEMENT_3D ( 'NONE', #6032, #9212, #9367 ) ;
#6781=FILL_AREA_STYLE_COLOUR ( '', #860 ) ;
#6787=ORIENTED_EDGE ( 'NONE', *, *, #2903, .F. ) ;
#6802=DIRECTION ( 'NONE',  ( -1.000000000000000000, -1.387778780781445676E-16, 0.000000000000000000 ) ) ;
#6814=CARTESIAN_POINT ( 'NONE',  ( -163.9101340986164246, -1.243481348857424562, 12.94061705906631055 ) ) ;
#6851=VERTEX_POINT ( 'NONE', #9258 ) ;
#6906=DIRECTION ( 'NONE',  ( 1.000000000000000000, 0.000000000000000000, 0.000000000000000000 ) ) ;
#6970=CARTESIAN_POINT ( 'NONE',  ( -158.0000000000000284, 17.99999999999999645, 2.204364238465235822E-15 ) ) ;
#6974=AXIS2_PLACEMENT_3D ( 'NONE', #8968, #1881, #4153 ) ;
#6987=VERTEX_POINT ( 'NONE', #3709 ) ;
#6993=DIRECTION ( 'NONE',  ( -1.000000000000000000, 4.575525868300071581E-16, 0.000000000000000000 ) ) ;
#7046=CARTESIAN_POINT ( 'NONE',  ( -158.0000000000000284, -6.938893903907228378E-15, 0.000000000000000000 ) ) ;
#7057=MANIFOLD_SOLID_BREP ( 'M4 Tapped Hole1', #4986 ) ;
#7068=ORIENTED_EDGE ( 'NONE', *, *, #8641, .F. ) ;
#7098=LINE ( 'NONE', #656, #1995 ) ;
#7114=COLOUR_RGB ( '', 0.31764706, 0.68627451, 0.89019608) ;
#7116=PRODUCT_DEFINITION_CONTEXT ( 'detailed design', #451, 'design' ) ;
#7140=CYLINDRICAL_SURFACE ( 'NONE', #9321, 13.00000000000000355 ) ;
#7200=CARTESIAN_POINT ( 'NONE',  ( -164.1743453116437763, -1.432625545945890311, 12.92095975507885441 ) ) ;
#7201=DIRECTION ( 'NONE',  ( 0.000000000000000000, -1.000000000000000000, 0.000000000000000000 ) ) ;
#7208=AXIS2_PLACEMENT_3D ( 'NONE', #5874, #9930, #5778 ) ;
#7275=ORIENTED_EDGE ( 'NONE', *, *, #6522, .F. ) ;
#7291=CARTESIAN_POINT ( 'NONE',  ( -163.3500000000000512, -1.154202410357457390E-14, 13.00000000000000355 ) ) ;
#7310=EDGE_LOOP ( 'NONE', ( #7275, #44 ) ) ;
#7331=VECTOR ( 'NONE', #1095, 999.9999999999998863 ) ;
#7363=DIRECTION ( 'NONE',  ( 1.000000000000000000, 0.000000000000000000, 0.000000000000000000 ) ) ;
#7387=CARTESIAN_POINT ( 'NONE',  ( -166.3117586239410457, 1.006644598837332039, 12.96127626484980233 ) ) ;
#7419=DIRECTION ( 'NONE',  ( 1.000000000000000000, 0.000000000000000000, 0.000000000000000000 ) ) ;
#7435=ADVANCED_FACE ( 'NONE', ( #2145 ), #6054, .T. ) ;
#7436=CONICAL_SURFACE ( 'NONE', #3988, 1.649999999999984812, 1.029744258676650093 ) ;
#7440=CARTESIAN_POINT ( 'NONE',  ( -166.4829340271541582, 0.7315032035247491793, 12.97978828447449828 ) ) ;
#7496=DIRECTION ( 'NONE',  ( -1.000000000000000000, -1.387778780781445676E-16, -0.000000000000000000 ) ) ;
#7553=DIRECTION ( 'NONE',  ( 0.000000000000000000, -1.000000000000000000, 0.000000000000000000 ) ) ;
#7591=VECTOR ( 'NONE', #5714, 999.9999999999998863 ) ;
#7602=AXIS2_PLACEMENT_3D ( 'NONE', #9502, #8511, #2310 ) ;
#7606=ORIENTED_EDGE ( 'NONE', *, *, #5317, .F. ) ;
#7669=CARTESIAN_POINT ( 'NONE',  ( -108.0000000000000426, 18.00000000000000355, 2.204364238465236217E-15 ) ) ;
#7670=CIRCLE ( 'NONE', #9154, 13.00000000000000355 ) ;
#7674=CYLINDRICAL_SURFACE ( 'NONE', #1826, 15.99999999999999645 ) ;
#7758=DIRECTION ( 'NONE',  ( -1.000000000000000000, -1.387778780781445676E-16, 0.000000000000000000 ) ) ;
#7781=DIRECTION ( 'NONE',  ( 0.000000000000000000, -1.000000000000000000, 0.000000000000000000 ) ) ;
#7782=AXIS2_PLACEMENT_3D ( 'NONE', #830, #5629, #6344 ) ;
#7789=EDGE_CURVE ( 'NONE', #9967, #5977, #7098, .T. ) ;
#7795=DIRECTION ( 'NONE',  ( 0.000000000000000000, -1.000000000000000000, 0.000000000000000000 ) ) ;
#7823=ORIENTED_EDGE ( 'NONE', *, *, #5286, .F. ) ;
#7825=DIRECTION ( 'NONE',  ( -0.000000000000000000, -0.000000000000000000, 1.000000000000000000 ) ) ;
#7869=VERTEX_POINT ( 'NONE', #3122 ) ;
#7871=CARTESIAN_POINT ( 'NONE',  ( -108.0000000000000426, 0.000000000000000000, 0.000000000000000000 ) ) ;
#7886=( LENGTH_UNIT ( ) NAMED_UNIT ( * ) SI_UNIT ( .MILLI., .METRE. ) );
#7888=PRODUCT_DEFINITION_FORMATION_WITH_SPECIFIED_SOURCE ( 'ANY', '', #5087, .NOT_KNOWN. ) ;
#7898=ORIENTED_EDGE ( 'NONE', *, *, #5911, .F. ) ;
#7923=TOROIDAL_SURFACE ( 'NONE', #4789, 11.00000000000000355, 2.000000000000000000 ) ;
#7940=( GEOMETRIC_REPRESENTATION_CONTEXT ( 3 ) GLOBAL_UNCERTAINTY_ASSIGNED_CONTEXT ( ( #5756 ) ) GLOBAL_UNIT_ASSIGNED_CONTEXT ( ( #7886, #8670, #10219 ) ) REPRESENTATION_CONTEXT ( 'NONE', 'WORKASPACE' ) );
#7965=CARTESIAN_POINT ( 'NONE',  ( -166.0896366705012781, 1.243800164630720406, 12.94059239432925068 ) ) ;
#7976=DIRECTION ( 'NONE',  ( 0.000000000000000000, 1.000000000000000000, 0.000000000000000000 ) ) ;
#7979=DIRECTION ( 'NONE',  ( -1.000000000000000000, -1.387778780781445676E-16, -0.000000000000000000 ) ) ;
#8016=DIRECTION ( 'NONE',  ( -1.000000000000000000, -1.387778780781445676E-16, -0.000000000000000000 ) ) ;
#8049=EDGE_LOOP ( 'NONE', ( #4661, #4539 ) ) ;
#8075=CARTESIAN_POINT ( 'NONE',  ( -163.9949573840844437, -1.313015978385311033, 12.93366173934393260 ) ) ;
#8085=FACE_OUTER_BOUND ( 'NONE', #4275, .T. ) ;
#8126=DIRECTION ( 'NONE',  ( 0.000000000000000000, 1.000000000000000000, 0.000000000000000000 ) ) ;
#8141=UNCERTAINTY_MEASURE_WITH_UNIT (LENGTH_MEASURE( 1.000000000000000082E-05 ), #1268, 'distance_accuracy_value', 'NONE');
#8160=FACE_BOUND ( 'NONE', #5531, .T. ) ;
#8199=ORIENTED_EDGE ( 'NONE', *, *, #2781, .T. ) ;
#8265=CARTESIAN_POINT ( 'NONE',  ( -166.6391998862286243, 0.2171903991958598068, 12.99861672450135330 ) ) ;
#8309=ORIENTED_EDGE ( 'NONE', *, *, #1508, .F. ) ;
#8364=ORIENTED_EDGE ( 'NONE', *, *, #2781, .F. ) ;
#8383=EDGE_CURVE ( 'NONE', #7869, #503, #1006, .T. ) ;
#8387=ORIENTED_EDGE ( 'NONE', *, *, #74, .T. ) ;
#8391=DIRECTION ( 'NONE',  ( 1.000000000000000000, 0.000000000000000000, 0.000000000000000000 ) ) ;
#8397=( LENGTH_UNIT ( ) NAMED_UNIT ( * ) SI_UNIT ( .MILLI., .METRE. ) );
#8404=ADVANCED_FACE ( 'NONE', ( #2239 ), #7674, .F. ) ;
#8413=VERTEX_POINT ( 'NONE', #2953 ) ;
#8424=DIRECTION ( 'NONE',  ( 1.000000000000000000, -4.575525868300071581E-16, -0.000000000000000000 ) ) ;
#8435=CIRCLE ( 'NONE', #4782, 18.00000000000000355 ) ;
#8448=FACE_OUTER_BOUND ( 'NONE', #662, .T. ) ;
#8449=DIRECTION ( 'NONE',  ( -1.000000000000000000, -1.387778780781445676E-16, -0.000000000000000000 ) ) ;
#8476=ORIENTED_EDGE ( 'NONE', *, *, #5748, .F. ) ;
#8494=DIRECTION ( 'NONE',  ( -1.000000000000000000, -1.387778780781445676E-16, -0.000000000000000000 ) ) ;
#8501=DIRECTION ( 'NONE',  ( -4.575525868300071581E-16, -1.000000000000000000, 0.000000000000000000 ) ) ;
#8508=SURFACE_SIDE_STYLE ('',( #1223 ) ) ;
#8511=DIRECTION ( 'NONE',  ( -1.000000000000000000, -1.387778780781445676E-16, -0.000000000000000000 ) ) ;
#8526=CARTESIAN_POINT ( 'NONE',  ( -165.0000000000000284, -1.734723475976807094E-15, 13.00000000000000355 ) ) ;
#8566=EDGE_CURVE ( 'NONE', #5977, #6851, #4964, .T. ) ;
#8575=ORIENTED_EDGE ( 'NONE', *, *, #5911, .T. ) ;
#8604=CIRCLE ( 'NONE', #6756, 15.99999999999999289 ) ;
#8617=CARTESIAN_POINT ( 'NONE',  ( -170.0000000000000284, -1.448262861947153525E-15, 0.000000000000000000 ) ) ;
#8620=AXIS2_PLACEMENT_3D ( 'NONE', #5249, #10013, #4541 ) ;
#8633=ORIENTED_EDGE ( 'NONE', *, *, #9584, .T. ) ;
#8641=EDGE_CURVE ( 'NONE', #8413, #6851, #3218, .T. ) ;
#8656=DIRECTION ( 'NONE',  ( -1.000000000000000000, -1.387778780781445676E-16, -0.000000000000000000 ) ) ;
#8670=( NAMED_UNIT ( * ) PLANE_ANGLE_UNIT ( ) SI_UNIT ( $, .RADIAN. ) );
#8706=FACE_OUTER_BOUND ( 'NONE', #5999, .T. ) ;
#8752=DIRECTION ( 'NONE',  ( 1.000000000000000000, -4.575525868300071581E-16, -0.000000000000000000 ) ) ;
#8802=CARTESIAN_POINT ( 'NONE',  ( -163.3607213683654606, 0.2164297246728172364, 12.99862687051388832 ) ) ;
#8837=DIRECTION ( 'NONE',  ( -4.575525868300071581E-16, -1.000000000000000000, 0.000000000000000000 ) ) ;
#8862=CARTESIAN_POINT ( 'NONE',  ( -166.0915134144852345, -1.242040127916074654, 12.94075629995628063 ) ) ;
#8896=ORIENTED_EDGE ( 'NONE', *, *, #1783, .T. ) ;
#8909=CARTESIAN_POINT ( 'NONE',  ( -166.6500000000000341, -1.532656777835077474E-15, 13.00000000000000355 ) ) ;
#8930=DIRECTION ( 'NONE',  ( 0.000000000000000000, 0.000000000000000000, 1.000000000000000000 ) ) ;
#8938=CIRCLE ( 'NONE', #1676, 15.99999999999999289 ) ;
#8939=EDGE_LOOP ( 'NONE', ( #8896, #5418 ) ) ;
#8940=MECHANICAL_DESIGN_GEOMETRIC_PRESENTATION_REPRESENTATION('',(#3152),#7940);
#8958=ADVANCED_BREP_SHAPE_REPRESENTATION ( '', ( #7057, #3995 ), #3161 ) ;
#8968=CARTESIAN_POINT ( 'NONE',  ( -168.0000000000000284, 11.00000000000000178, 1.347111479062088799E-15 ) ) ;
#8970=EDGE_CURVE ( 'NONE', #9396, #10190, #833, .T. ) ;
#8996=VECTOR ( 'NONE', #4235, 1000.000000000000000 ) ;
#9041=ORIENTED_EDGE ( 'NONE', *, *, #9306, .T. ) ;
#9077=DIRECTION ( 'NONE',  ( -1.000000000000000000, 4.575525868300071581E-16, 0.000000000000000000 ) ) ;
#9104=CARTESIAN_POINT ( 'NONE',  ( -166.5657114886604120, 0.5317309469415117951, 12.98950588154195351 ) ) ;
#9110=CARTESIAN_POINT ( 'NONE',  ( -158.0000000000000284, -18.00000000000001066, 0.000000000000000000 ) ) ;
#9116=VERTEX_POINT ( 'NONE', #9110 ) ;
#9154=AXIS2_PLACEMENT_3D ( 'NONE', #1248, #4454, #7553 ) ;
#9158=CARTESIAN_POINT ( 'NONE',  ( -163.3500000000000512, -1.154202410357457390E-14, 13.00000000000000355 ) ) ;
#9178=EDGE_LOOP ( 'NONE', ( #3598, #9997, #726, #4312 ) ) ;
#9212=DIRECTION ( 'NONE',  ( -1.000000000000000000, -1.387778780781445676E-16, -0.000000000000000000 ) ) ;
#9216=DIRECTION ( 'NONE',  ( 1.000000000000000000, -4.575525868300071581E-16, -0.000000000000000000 ) ) ;
#9235=( NAMED_UNIT ( * ) PLANE_ANGLE_UNIT ( ) SI_UNIT ( $, .RADIAN. ) );
#9240=EDGE_LOOP ( 'NONE', ( #10150, #6633 ) ) ;
#9258=CARTESIAN_POINT ( 'NONE',  ( -156.0000000000000284, 15.99999999999999289, 1.959434878635764737E-15 ) ) ;
#9306=EDGE_CURVE ( 'NONE', #6851, #5977, #5288, .T. ) ;
#9321=AXIS2_PLACEMENT_3D ( 'NONE', #4044, #4192, #9679 ) ;
#9349=EDGE_CURVE ( 'NONE', #5718, #6987, #181, .T. ) ;
#9367=DIRECTION ( 'NONE',  ( 0.000000000000000000, -1.000000000000000000, 0.000000000000000000 ) ) ;
#9396=VERTEX_POINT ( 'NONE', #5066 ) ;
#9429=CIRCLE ( 'NONE', #7602, 18.00000000000000355 ) ;
#9443=CARTESIAN_POINT ( 'NONE',  ( -170.0000000000000284, -11.00000000000000533, 0.000000000000000000 ) ) ;
#9463=ADVANCED_FACE ( 'NONE', ( #2734 ), #7436, .F. ) ;
#9475=DIRECTION ( 'NONE',  ( 1.387778780781445676E-16, -1.000000000000000000, 0.000000000000000000 ) ) ;
#9477=CARTESIAN_POINT ( 'NONE',  ( -108.0000000000000426, -15.99999999999999289, 0.000000000000000000 ) ) ;
#9478=ORIENTED_EDGE ( 'NONE', *, *, #6620, .F. ) ;
#9502=CARTESIAN_POINT ( 'NONE',  ( -108.0000000000000426, 0.000000000000000000, 0.000000000000000000 ) ) ;
#9506=PRESENTATION_STYLE_ASSIGNMENT (( #6324 ) ) ;
#9529=CARTESIAN_POINT ( 'NONE',  ( -165.7311118698760026, 1.483131377360883185, 12.91518709242523855 ) ) ;
#9539=CARTESIAN_POINT ( 'NONE',  ( -165.1102640658071437, -1.649921999561606567, 12.89487329916352465 ) ) ;
#9562=FACE_OUTER_BOUND ( 'NONE', #4573, .T. ) ;
#9577=CARTESIAN_POINT ( 'NONE',  ( -166.6500000000000341, -1.532656754117495520E-15, 13.00000000000000355 ) ) ;
#9584=EDGE_CURVE ( 'NONE', #8413, #9967, #8604, .T. ) ;
#9652=EDGE_CURVE ( 'NONE', #7869, #1613, #685, .T. ) ;
#9657=FILL_AREA_STYLE ('',( #3342 ) ) ;
#9679=DIRECTION ( 'NONE',  ( 0.000000000000000000, 1.000000000000000000, 0.000000000000000000 ) ) ;
#9685=LINE ( 'NONE', #6410, #5870 ) ;
#9697=ORIENTED_EDGE ( 'NONE', *, *, #8641, .T. ) ;
#9726=ORIENTED_EDGE ( 'NONE', *, *, #3204, .T. ) ;
#9770=AXIS2_PLACEMENT_3D ( 'NONE', #6649, #472, #6744 ) ;
#9776=MECHANICAL_DESIGN_GEOMETRIC_PRESENTATION_REPRESENTATION('',(#4486),#1352);
#9837=ORIENTED_EDGE ( 'NONE', *, *, #7789, .T. ) ;
#9871=ADVANCED_FACE ( 'NONE', ( #152, #781 ), #3986, .F. ) ;
#9873=ORIENTED_EDGE ( 'NONE', *, *, #6620, .T. ) ;
#9875=CARTESIAN_POINT ( 'NONE',  ( -158.0000000000000284, 12.99999999999999645, 0.000000000000000000 ) ) ;
#9898=CARTESIAN_POINT ( 'NONE',  ( -158.0000000000000284, 12.99999999999999822, 0.000000000000000000 ) ) ;
#9900=FACE_OUTER_BOUND ( 'NONE', #6642, .T. ) ;
#9910=( NAMED_UNIT ( * ) PLANE_ANGLE_UNIT ( ) SI_UNIT ( $, .RADIAN. ) );
#9916=EDGE_LOOP ( 'NONE', ( #6787, #1905, #6335, #3689 ) ) ;
#9930=DIRECTION ( 'NONE',  ( -1.000000000000000000, -1.387778780781445676E-16, -0.000000000000000000 ) ) ;
#9950=ORIENTED_EDGE ( 'NONE', *, *, #8970, .T. ) ;
#9967=VERTEX_POINT ( 'NONE', #9477 ) ;
#9997=ORIENTED_EDGE ( 'NONE', *, *, #9349, .T. ) ;
#10001=CYLINDRICAL_SURFACE ( 'NONE', #3190, 1.649999999999984812 ) ;
#10013=DIRECTION ( 'NONE',  ( -1.000000000000000000, -1.387778780781445676E-16, -0.000000000000000000 ) ) ;
#10073=AXIS2_PLACEMENT_3D ( 'NONE', #4607, #7758, #9475 ) ;
#10092=TOROIDAL_SURFACE ( 'NONE', #3153, 11.00000000000000355, 2.000000000000000000 ) ;
#10115=LINE ( 'NONE', #5556, #4301 ) ;
#10132=PLANE ( 'NONE',  #10073 ) ;
#10146=CARTESIAN_POINT ( 'NONE',  ( -156.0000000000000284, -6.661338147750945553E-15, 0.000000000000000000 ) ) ;
#10150=ORIENTED_EDGE ( 'NONE', *, *, #8566, .F. ) ;
#10155=APPLICATION_CONTEXT ( 'automotive_design' ) ;
#10163=DIRECTION ( 'NONE',  ( -1.000000000000000000, 4.575525868300071581E-16, 0.000000000000000000 ) ) ;
#10170=PRODUCT_CONTEXT ( 'NONE', #10155, 'mechanical' ) ;
#10190=VERTEX_POINT ( 'NONE', #3394 ) ;
#10219=( NAMED_UNIT ( * ) SI_UNIT ( $, .STERADIAN. ) SOLID_ANGLE_UNIT ( ) );
ENDSEC;
END-ISO-10303-21;
